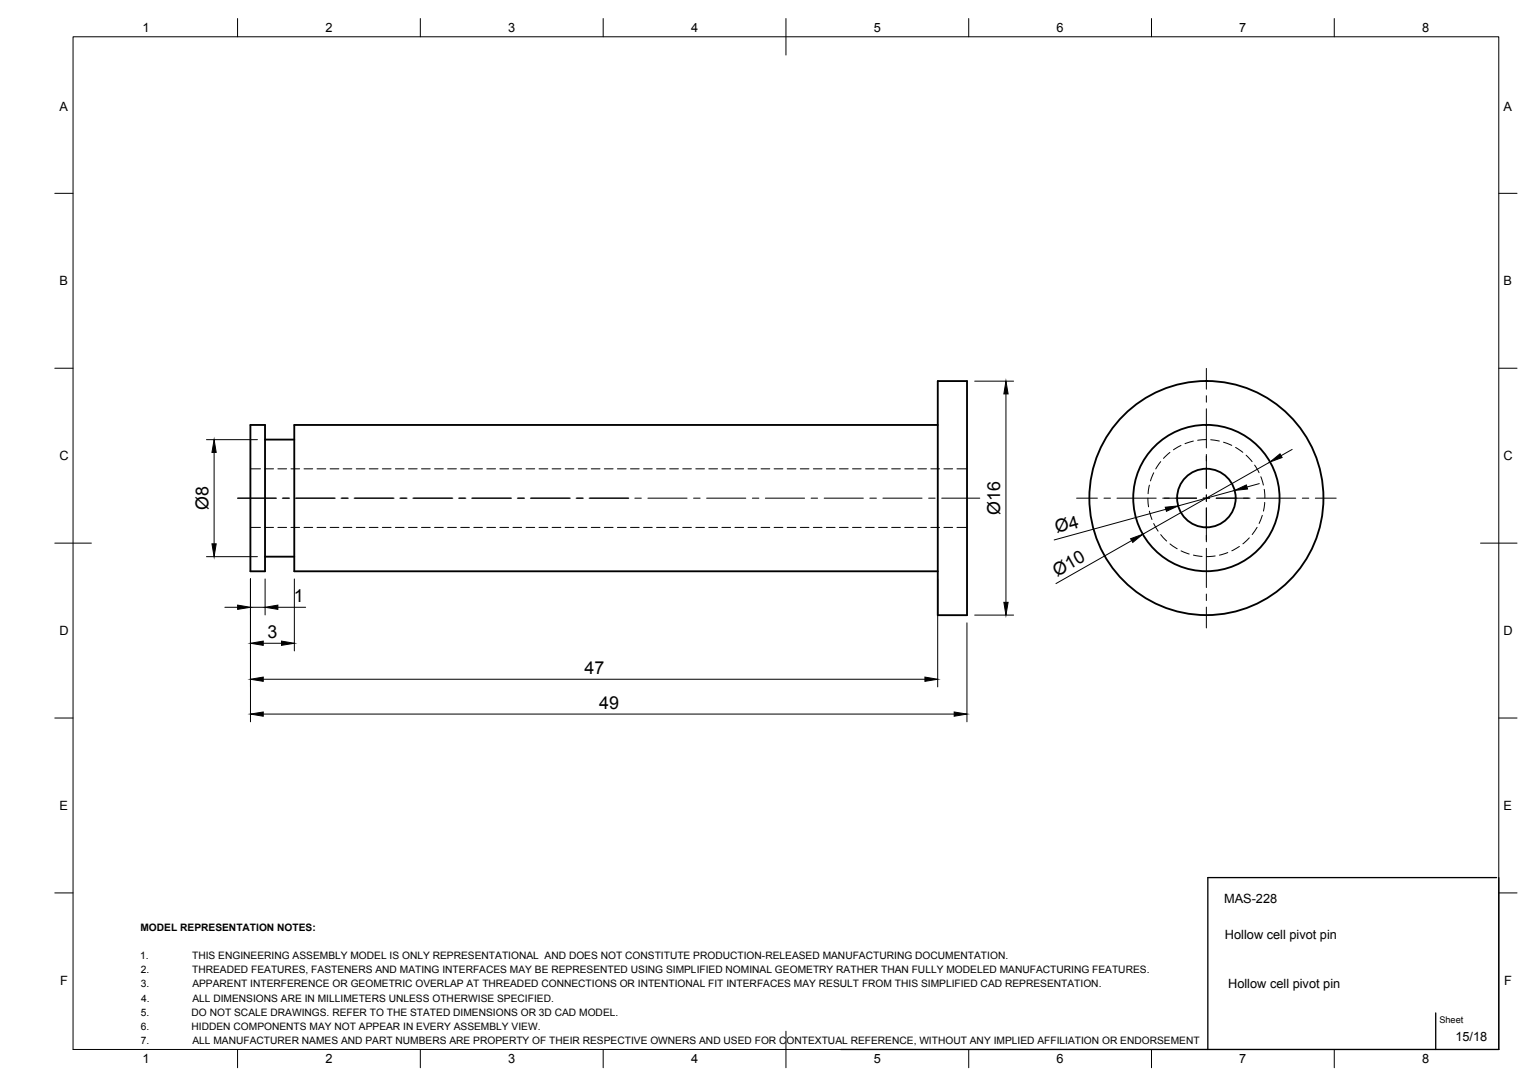
ISO-10303-21;
HEADER;
/* Generated by software containing ST-Developer
 * from STEP Tools, Inc. (www.steptools.com) 
 */

FILE_DESCRIPTION(
/* description */ ('Independent Peaucellier-Lipkin straight-line linkage. Radius arms 100
 mm, inversion-cell links 60 mm, crank radius and fixed-pivot spacing 
32 mm. Inversion constant 6400 mm squared, nominal output straight lin
e X=100 mm. Overhead bearing bridge clears the layered moving links. N
o accuracy or load rating assigned.'),
/* implementation_level */ '2;1');

FILE_NAME(
/* name */ 'Hollow cell pivot pin.step',
/* time_stamp */ '2026-11-09T18:06:16-08:00',
/* author */ (''),
/* organization */ (''),
/* preprocessor_version */ 'ST-DEVELOPER v20.2',
/* originating_system */ 'Autodesk Translation Framework v15.17.0.0',
/* authorisation */ '');

FILE_SCHEMA (('AUTOMOTIVE_DESIGN { 1 0 10303 214 3 1 1 }'));
ENDSEC;

DATA;
#10=MECHANICAL_DESIGN_GEOMETRIC_PRESENTATION_REPRESENTATION('',(#292),#3581);
#258=SHAPE_REPRESENTATION_RELATIONSHIP('SRR','None',#3692,#275);
#275=ADVANCED_BREP_SHAPE_REPRESENTATION('',(#309),#3574);
#292=STYLED_ITEM('',(#3782),#309);
#309=MANIFOLD_SOLID_BREP('Body1',#1878);
#350=FACE_BOUND('',#643,.T.);
#351=FACE_BOUND('',#645,.T.);
#352=FACE_BOUND('',#648,.T.);
#353=FACE_BOUND('',#651,.T.);
#354=FACE_BOUND('',#655,.T.);
#404=PLANE('',#2221);
#405=PLANE('',#2223);
#406=PLANE('',#2227);
#407=PLANE('',#2232);
#408=PLANE('',#2237);
#496=FACE_OUTER_BOUND('',#641,.T.);
#497=FACE_OUTER_BOUND('',#642,.T.);
#498=FACE_OUTER_BOUND('',#644,.T.);
#499=FACE_OUTER_BOUND('',#646,.T.);
#500=FACE_OUTER_BOUND('',#647,.T.);
#501=FACE_OUTER_BOUND('',#649,.T.);
#502=FACE_OUTER_BOUND('',#650,.T.);
#503=FACE_OUTER_BOUND('',#652,.T.);
#504=FACE_OUTER_BOUND('',#653,.T.);
#505=FACE_OUTER_BOUND('',#654,.T.);
#641=EDGE_LOOP('',(#1586,#1587,#1588,#1589));
#642=EDGE_LOOP('',(#1590));
#643=EDGE_LOOP('',(#1591));
#644=EDGE_LOOP('',(#1592));
#645=EDGE_LOOP('',(#1593));
#646=EDGE_LOOP('',(#1594,#1595,#1596,#1597));
#647=EDGE_LOOP('',(#1598));
#648=EDGE_LOOP('',(#1599));
#649=EDGE_LOOP('',(#1600,#1601,#1602,#1603));
#650=EDGE_LOOP('',(#1604));
#651=EDGE_LOOP('',(#1605));
#652=EDGE_LOOP('',(#1606,#1607,#1608,#1609));
#653=EDGE_LOOP('',(#1610,#1611,#1612,#1613));
#654=EDGE_LOOP('',(#1614));
#655=EDGE_LOOP('',(#1615));
#768=LINE('',#3341,#866);
#769=LINE('',#3352,#867);
#770=LINE('',#3360,#868);
#771=LINE('',#3368,#869);
#772=LINE('',#3370,#870);
#866=VECTOR('',#2726,4.);
#867=VECTOR('',#2741,5.);
#868=VECTOR('',#2750,8.);
#869=VECTOR('',#2761,2.);
#870=VECTOR('',#2764,5.);
#953=CIRCLE('',#2219,4.);
#954=CIRCLE('',#2220,4.);
#955=CIRCLE('',#2222,5.);
#956=CIRCLE('',#2224,5.);
#957=CIRCLE('',#2226,5.);
#958=CIRCLE('',#2228,8.);
#959=CIRCLE('',#2229,5.);
#960=CIRCLE('',#2231,8.);
#961=CIRCLE('',#2233,2.);
#962=CIRCLE('',#2235,2.);
#1079=VERTEX_POINT('',#3338);
#1080=VERTEX_POINT('',#3340);
#1081=VERTEX_POINT('',#3344);
#1082=VERTEX_POINT('',#3347);
#1083=VERTEX_POINT('',#3350);
#1084=VERTEX_POINT('',#3354);
#1085=VERTEX_POINT('',#3356);
#1086=VERTEX_POINT('',#3359);
#1087=VERTEX_POINT('',#3363);
#1088=VERTEX_POINT('',#3366);
#1255=EDGE_CURVE('',#1079,#1079,#953,.T.);
#1256=EDGE_CURVE('',#1079,#1080,#768,.T.);
#1257=EDGE_CURVE('',#1080,#1080,#954,.T.);
#1258=EDGE_CURVE('',#1081,#1081,#955,.T.);
#1259=EDGE_CURVE('',#1082,#1082,#956,.T.);
#1260=EDGE_CURVE('',#1083,#1083,#957,.T.);
#1261=EDGE_CURVE('',#1083,#1082,#769,.T.);
#1262=EDGE_CURVE('',#1084,#1084,#958,.T.);
#1263=EDGE_CURVE('',#1085,#1085,#959,.T.);
#1264=EDGE_CURVE('',#1084,#1086,#770,.T.);
#1265=EDGE_CURVE('',#1086,#1086,#960,.T.);
#1266=EDGE_CURVE('',#1087,#1087,#961,.T.);
#1267=EDGE_CURVE('',#1088,#1088,#962,.T.);
#1268=EDGE_CURVE('',#1088,#1087,#771,.T.);
#1269=EDGE_CURVE('',#1081,#1085,#772,.T.);
#1586=ORIENTED_EDGE('',*,*,#1255,.T.);
#1587=ORIENTED_EDGE('',*,*,#1256,.T.);
#1588=ORIENTED_EDGE('',*,*,#1257,.F.);
#1589=ORIENTED_EDGE('',*,*,#1256,.F.);
#1590=ORIENTED_EDGE('',*,*,#1258,.F.);
#1591=ORIENTED_EDGE('',*,*,#1255,.F.);
#1592=ORIENTED_EDGE('',*,*,#1259,.F.);
#1593=ORIENTED_EDGE('',*,*,#1257,.T.);
#1594=ORIENTED_EDGE('',*,*,#1260,.F.);
#1595=ORIENTED_EDGE('',*,*,#1261,.T.);
#1596=ORIENTED_EDGE('',*,*,#1259,.T.);
#1597=ORIENTED_EDGE('',*,*,#1261,.F.);
#1598=ORIENTED_EDGE('',*,*,#1262,.T.);
#1599=ORIENTED_EDGE('',*,*,#1263,.F.);
#1600=ORIENTED_EDGE('',*,*,#1262,.F.);
#1601=ORIENTED_EDGE('',*,*,#1264,.T.);
#1602=ORIENTED_EDGE('',*,*,#1265,.T.);
#1603=ORIENTED_EDGE('',*,*,#1264,.F.);
#1604=ORIENTED_EDGE('',*,*,#1265,.F.);
#1605=ORIENTED_EDGE('',*,*,#1266,.F.);
#1606=ORIENTED_EDGE('',*,*,#1267,.F.);
#1607=ORIENTED_EDGE('',*,*,#1268,.T.);
#1608=ORIENTED_EDGE('',*,*,#1266,.T.);
#1609=ORIENTED_EDGE('',*,*,#1268,.F.);
#1610=ORIENTED_EDGE('',*,*,#1258,.T.);
#1611=ORIENTED_EDGE('',*,*,#1269,.T.);
#1612=ORIENTED_EDGE('',*,*,#1263,.T.);
#1613=ORIENTED_EDGE('',*,*,#1269,.F.);
#1614=ORIENTED_EDGE('',*,*,#1260,.T.);
#1615=ORIENTED_EDGE('',*,*,#1267,.T.);
#1739=CYLINDRICAL_SURFACE('',#2218,4.);
#1740=CYLINDRICAL_SURFACE('',#2225,5.);
#1741=CYLINDRICAL_SURFACE('',#2230,8.);
#1742=CYLINDRICAL_SURFACE('',#2234,2.);
#1743=CYLINDRICAL_SURFACE('',#2236,5.);
#1828=ADVANCED_FACE('',(#496),#1739,.T.);
#1829=ADVANCED_FACE('',(#497,#350),#404,.F.);
#1830=ADVANCED_FACE('',(#498,#351),#405,.F.);
#1831=ADVANCED_FACE('',(#499),#1740,.T.);
#1832=ADVANCED_FACE('',(#500,#352),#406,.T.);
#1833=ADVANCED_FACE('',(#501),#1741,.T.);
#1834=ADVANCED_FACE('',(#502,#353),#407,.F.);
#1835=ADVANCED_FACE('',(#503),#1742,.F.);
#1836=ADVANCED_FACE('',(#504),#1743,.T.);
#1837=ADVANCED_FACE('',(#505,#354),#408,.T.);
#1878=CLOSED_SHELL('',(#1828,#1829,#1830,#1831,#1832,#1833,#1834,#1835,
#1836,#1837));
#2217=AXIS2_PLACEMENT_3D('',#3336,#2720,#2721);
#2218=AXIS2_PLACEMENT_3D('',#3337,#2722,#2723);
#2219=AXIS2_PLACEMENT_3D('',#3339,#2724,#2725);
#2220=AXIS2_PLACEMENT_3D('',#3342,#2727,#2728);
#2221=AXIS2_PLACEMENT_3D('',#3343,#2729,#2730);
#2222=AXIS2_PLACEMENT_3D('',#3345,#2731,#2732);
#2223=AXIS2_PLACEMENT_3D('',#3346,#2733,#2734);
#2224=AXIS2_PLACEMENT_3D('',#3348,#2735,#2736);
#2225=AXIS2_PLACEMENT_3D('',#3349,#2737,#2738);
#2226=AXIS2_PLACEMENT_3D('',#3351,#2739,#2740);
#2227=AXIS2_PLACEMENT_3D('',#3353,#2742,#2743);
#2228=AXIS2_PLACEMENT_3D('',#3355,#2744,#2745);
#2229=AXIS2_PLACEMENT_3D('',#3357,#2746,#2747);
#2230=AXIS2_PLACEMENT_3D('',#3358,#2748,#2749);
#2231=AXIS2_PLACEMENT_3D('',#3361,#2751,#2752);
#2232=AXIS2_PLACEMENT_3D('',#3362,#2753,#2754);
#2233=AXIS2_PLACEMENT_3D('',#3364,#2755,#2756);
#2234=AXIS2_PLACEMENT_3D('',#3365,#2757,#2758);
#2235=AXIS2_PLACEMENT_3D('',#3367,#2759,#2760);
#2236=AXIS2_PLACEMENT_3D('',#3369,#2762,#2763);
#2237=AXIS2_PLACEMENT_3D('',#3371,#2765,#2766);
#2720=DIRECTION('axis',(0.,0.,1.));
#2721=DIRECTION('refdir',(1.,0.,0.));
#2722=DIRECTION('center_axis',(0.,0.,1.));
#2723=DIRECTION('ref_axis',(1.,0.,0.));
#2724=DIRECTION('center_axis',(0.,0.,1.));
#2725=DIRECTION('ref_axis',(1.,0.,0.));
#2726=DIRECTION('',(0.,0.,1.));
#2727=DIRECTION('center_axis',(0.,0.,1.));
#2728=DIRECTION('ref_axis',(1.,0.,0.));
#2729=DIRECTION('center_axis',(0.,0.,-1.));
#2730=DIRECTION('ref_axis',(-1.,0.,0.));
#2731=DIRECTION('center_axis',(0.,0.,-1.));
#2732=DIRECTION('ref_axis',(1.,0.,0.));
#2733=DIRECTION('center_axis',(0.,0.,1.));
#2734=DIRECTION('ref_axis',(1.,0.,0.));
#2735=DIRECTION('center_axis',(0.,0.,1.));
#2736=DIRECTION('ref_axis',(1.,0.,0.));
#2737=DIRECTION('center_axis',(0.,0.,1.));
#2738=DIRECTION('ref_axis',(1.,0.,0.));
#2739=DIRECTION('center_axis',(0.,0.,1.));
#2740=DIRECTION('ref_axis',(1.,0.,0.));
#2741=DIRECTION('',(0.,0.,-1.));
#2742=DIRECTION('center_axis',(0.,0.,1.));
#2743=DIRECTION('ref_axis',(1.,0.,0.));
#2744=DIRECTION('center_axis',(0.,0.,1.));
#2745=DIRECTION('ref_axis',(1.,0.,0.));
#2746=DIRECTION('center_axis',(0.,0.,1.));
#2747=DIRECTION('ref_axis',(1.,0.,0.));
#2748=DIRECTION('center_axis',(0.,0.,1.));
#2749=DIRECTION('ref_axis',(1.,0.,0.));
#2750=DIRECTION('',(0.,0.,-1.));
#2751=DIRECTION('center_axis',(0.,0.,1.));
#2752=DIRECTION('ref_axis',(1.,0.,0.));
#2753=DIRECTION('center_axis',(0.,0.,1.));
#2754=DIRECTION('ref_axis',(1.,0.,0.));
#2755=DIRECTION('center_axis',(0.,0.,-1.));
#2756=DIRECTION('ref_axis',(1.,0.,0.));
#2757=DIRECTION('center_axis',(0.,0.,1.));
#2758=DIRECTION('ref_axis',(1.,0.,0.));
#2759=DIRECTION('center_axis',(0.,0.,-1.));
#2760=DIRECTION('ref_axis',(1.,0.,0.));
#2761=DIRECTION('',(0.,0.,-1.));
#2762=DIRECTION('center_axis',(0.,0.,1.));
#2763=DIRECTION('ref_axis',(1.,0.,0.));
#2764=DIRECTION('',(0.,0.,-1.));
#2765=DIRECTION('center_axis',(0.,0.,1.));
#2766=DIRECTION('ref_axis',(1.,0.,0.));
#3336=CARTESIAN_POINT('',(0.,0.,0.));
#3337=CARTESIAN_POINT('Origin',(0.,0.,45.));
#3338=CARTESIAN_POINT('',(-4.,-4.89858719658941E-16,44.));
#3339=CARTESIAN_POINT('Origin',(0.,0.,44.));
#3340=CARTESIAN_POINT('',(-4.,-4.89858719658941E-16,46.));
#3341=CARTESIAN_POINT('',(-4.,-4.89858719658941E-16,45.));
#3342=CARTESIAN_POINT('Origin',(0.,0.,46.));
#3343=CARTESIAN_POINT('Origin',(8.,0.,44.));
#3344=CARTESIAN_POINT('',(-5.,6.12323399573677E-16,44.));
#3345=CARTESIAN_POINT('Origin',(0.,0.,44.));
#3346=CARTESIAN_POINT('Origin',(4.,0.,46.));
#3347=CARTESIAN_POINT('',(-5.,-6.12323399573677E-16,46.));
#3348=CARTESIAN_POINT('Origin',(0.,0.,46.));
#3349=CARTESIAN_POINT('Origin',(0.,0.,0.));
#3350=CARTESIAN_POINT('',(-5.,-6.12323399573677E-16,47.));
#3351=CARTESIAN_POINT('Origin',(0.,0.,47.));
#3352=CARTESIAN_POINT('',(-5.,-6.12323399573677E-16,0.));
#3353=CARTESIAN_POINT('Origin',(0.,0.,0.));
#3354=CARTESIAN_POINT('',(-8.,-9.79717439317883E-16,0.));
#3355=CARTESIAN_POINT('Origin',(0.,0.,0.));
#3356=CARTESIAN_POINT('',(-5.,-6.12323399573677E-16,0.));
#3357=CARTESIAN_POINT('Origin',(0.,0.,0.));
#3358=CARTESIAN_POINT('Origin',(0.,0.,-2.));
#3359=CARTESIAN_POINT('',(-8.,-9.79717439317883E-16,-2.));
#3360=CARTESIAN_POINT('',(-8.,-9.79717439317883E-16,-2.));
#3361=CARTESIAN_POINT('Origin',(0.,0.,-2.));
#3362=CARTESIAN_POINT('Origin',(0.,0.,-2.));
#3363=CARTESIAN_POINT('',(-2.,-2.44929359829471E-16,-2.));
#3364=CARTESIAN_POINT('Origin',(0.,0.,-2.));
#3365=CARTESIAN_POINT('Origin',(0.,0.,0.));
#3366=CARTESIAN_POINT('',(-2.,-2.44929359829471E-16,47.));
#3367=CARTESIAN_POINT('Origin',(0.,0.,47.));
#3368=CARTESIAN_POINT('',(-2.,-2.44929359829471E-16,0.));
#3369=CARTESIAN_POINT('Origin',(0.,0.,0.));
#3370=CARTESIAN_POINT('',(-5.,-6.12323399573677E-16,0.));
#3371=CARTESIAN_POINT('Origin',(0.,0.,47.));
#3555=UNCERTAINTY_MEASURE_WITH_UNIT(LENGTH_MEASURE(0.01),#3582,
'DISTANCE_ACCURACY_VALUE',
'Maximum model space distance between geometric entities at asserted c
onnectivities');
#3562=UNCERTAINTY_MEASURE_WITH_UNIT(LENGTH_MEASURE(0.01),#3582,
'DISTANCE_ACCURACY_VALUE',
'Maximum model space distance between geometric entities at asserted c
onnectivities');
#3574=(
GEOMETRIC_REPRESENTATION_CONTEXT(3)
GLOBAL_UNCERTAINTY_ASSIGNED_CONTEXT((#3555))
GLOBAL_UNIT_ASSIGNED_CONTEXT((#3582,#3584,#3585))
REPRESENTATION_CONTEXT('','3D')
);
#3581=(
GEOMETRIC_REPRESENTATION_CONTEXT(3)
GLOBAL_UNCERTAINTY_ASSIGNED_CONTEXT((#3562))
GLOBAL_UNIT_ASSIGNED_CONTEXT((#3582,#3584,#3585))
REPRESENTATION_CONTEXT('','3D')
);
#3582=(
LENGTH_UNIT()
NAMED_UNIT(*)
SI_UNIT(.MILLI.,.METRE.)
);
#3584=(
NAMED_UNIT(*)
PLANE_ANGLE_UNIT()
SI_UNIT($,.RADIAN.)
);
#3585=(
NAMED_UNIT(*)
SI_UNIT($,.STERADIAN.)
SOLID_ANGLE_UNIT()
);
#3597=SHAPE_DEFINITION_REPRESENTATION(#3615,#3692);
#3615=PRODUCT_DEFINITION_SHAPE('',$,#3711);
#3692=SHAPE_REPRESENTATION('',(#2217),#3574);
#3699=PRODUCT_DEFINITION_CONTEXT('part definition',#3755,'design');
#3711=PRODUCT_DEFINITION('Hollow cell pivot pin',
'Hollow cell pivot pin',#3729,#3699);
#3729=PRODUCT_DEFINITION_FORMATION('',$,#3768);
#3755=APPLICATION_CONTEXT(
'Core Data for Automotive Mechanical Design Process');
#3756=PRODUCT_CONTEXT('part definition',#3755,'mechanical');
#3768=PRODUCT('Hollow cell pivot pin','Hollow cell pivot pin',$,(#3756));
#3782=PRESENTATION_STYLE_ASSIGNMENT((#3795));
#3795=SURFACE_STYLE_USAGE(.BOTH.,#3808);
#3808=SURFACE_SIDE_STYLE('',(#3821));
#3821=SURFACE_STYLE_FILL_AREA(#3834);
#3834=FILL_AREA_STYLE('Pivot gray',(#3847));
#3847=FILL_AREA_STYLE_COLOUR('Pivot gray',#3860);
#3860=COLOUR_RGB('Pivot gray',0.407843137254902,0.447058823529412,0.498039215686275);
ENDSEC;
END-ISO-10303-21;
